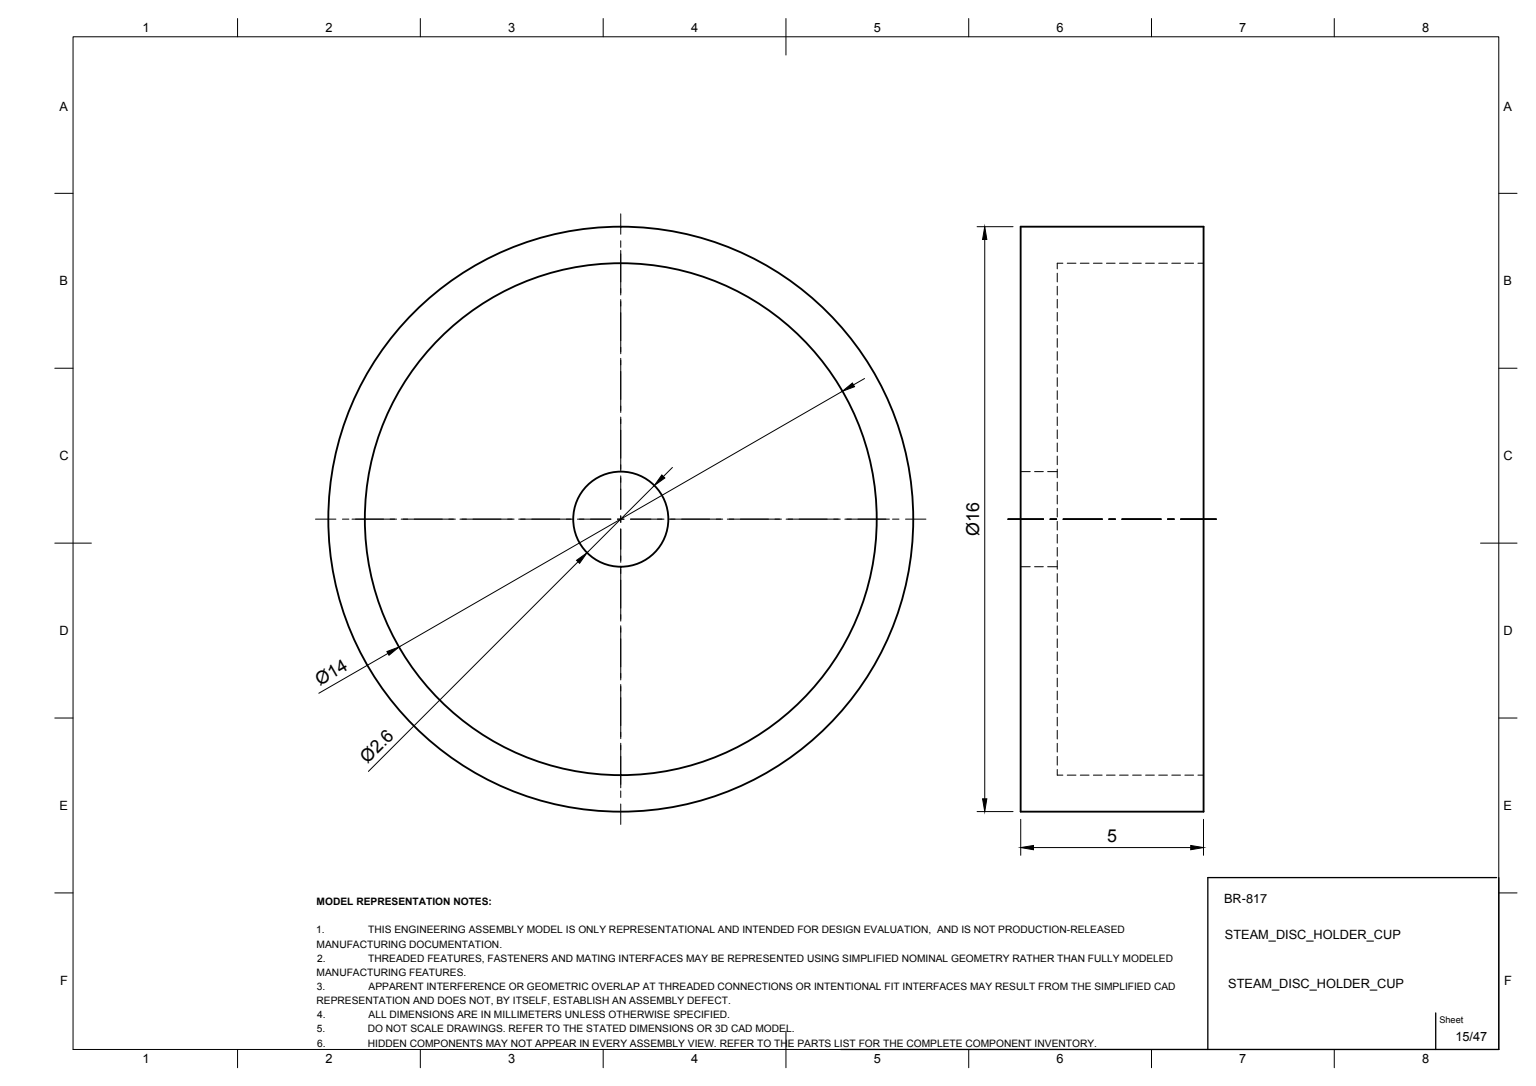
ISO-10303-21;
HEADER;
FILE_DESCRIPTION((''),'2;1');
FILE_NAME('STEAM_DISC_HOLDER_CUP.step','2026-10-01T22:07:29-07:00',(''),(''),'','','');
FILE_SCHEMA (('AUTOMOTIVE_DESIGN { 1 0 10303 214 3 1 1 }'));
ENDSEC;
DATA;
#10=MECHANICAL_DESIGN_GEOMETRIC_PRESENTATION_REPRESENTATION('',(#549),#15484);
#479=SHAPE_REPRESENTATION_RELATIONSHIP('SRR','None',#15628,#514) ;
#514=ADVANCED_BREP_SHAPE_REPRESENTATION('',(#591),#15452) ;
#549=STYLED_ITEM('',(#15834),#591) ;
#591=MANIFOLD_SOLID_BREP('STEAM_DISC_HOLDER_CUP',#8258) ;
#657=CYLINDRICAL_SURFACE('',#8871,0.13) ;
#658=CYLINDRICAL_SURFACE('',#8874,0.7) ;
#659=CYLINDRICAL_SURFACE('',#8879,0.8) ;
#849=FACE_BOUND('',#2016,.T.) ;
#850=FACE_BOUND('',#2019,.T.) ;
#851=FACE_BOUND('',#2021,.T.) ;
#948=CIRCLE('',#8872,0.13) ;
#949=CIRCLE('',#8873,0.13) ;
#950=CIRCLE('',#8875,0.7) ;
#951=CIRCLE('',#8876,0.7) ;
#952=CIRCLE('',#8878,0.8) ;
#953=CIRCLE('',#8880,0.8) ;
#1474=FACE_OUTER_BOUND('',#2013,.T.) ;
#1475=FACE_OUTER_BOUND('',#2014,.T.) ;
#1476=FACE_OUTER_BOUND('',#2015,.T.) ;
#1477=FACE_OUTER_BOUND('',#2017,.T.) ;
#1478=FACE_OUTER_BOUND('',#2018,.T.) ;
#1479=FACE_OUTER_BOUND('',#2020,.T.) ;
#2013=EDGE_LOOP('',(#5743,#5744,#5745,#5746)) ;
#2014=EDGE_LOOP('',(#5747,#5748,#5749,#5750)) ;
#2015=EDGE_LOOP('',(#5751)) ;
#2016=EDGE_LOOP('',(#5752)) ;
#2017=EDGE_LOOP('',(#5753,#5754,#5755,#5756)) ;
#2018=EDGE_LOOP('',(#5757)) ;
#2019=EDGE_LOOP('',(#5758)) ;
#2020=EDGE_LOOP('',(#5759)) ;
#2021=EDGE_LOOP('',(#5760)) ;
#2612=LINE('',#13407,#3086) ;
#2613=LINE('',#13413,#3087) ;
#2614=LINE('',#13420,#3088) ;
#3086=VECTOR('',#10479,0.13) ;
#3087=VECTOR('',#10486,0.7) ;
#3088=VECTOR('',#10495,0.8) ;
#3545=VERTEX_POINT('',#13404) ;
#3546=VERTEX_POINT('',#13406) ;
#3547=VERTEX_POINT('',#13410) ;
#3548=VERTEX_POINT('',#13412) ;
#3549=VERTEX_POINT('',#13416) ;
#3550=VERTEX_POINT('',#13419) ;
#4376=EDGE_CURVE('',#3545,#3545,#948,.T.) ;
#4377=EDGE_CURVE('',#3545,#3546,#2612,.T.) ;
#4378=EDGE_CURVE('',#3546,#3546,#949,.T.) ;
#4379=EDGE_CURVE('',#3547,#3547,#950,.T.) ;
#4380=EDGE_CURVE('',#3547,#3548,#2613,.T.) ;
#4381=EDGE_CURVE('',#3548,#3548,#951,.T.) ;
#4382=EDGE_CURVE('',#3549,#3549,#952,.T.) ;
#4383=EDGE_CURVE('',#3549,#3550,#2614,.T.) ;
#4384=EDGE_CURVE('',#3550,#3550,#953,.T.) ;
#5743=ORIENTED_EDGE('',*,*,#4376,.F.) ;
#5744=ORIENTED_EDGE('',*,*,#4377,.T.) ;
#5745=ORIENTED_EDGE('',*,*,#4378,.F.) ;
#5746=ORIENTED_EDGE('',*,*,#4377,.F.) ;
#5747=ORIENTED_EDGE('',*,*,#4379,.F.) ;
#5748=ORIENTED_EDGE('',*,*,#4380,.T.) ;
#5749=ORIENTED_EDGE('',*,*,#4381,.F.) ;
#5750=ORIENTED_EDGE('',*,*,#4380,.F.) ;
#5751=ORIENTED_EDGE('',*,*,#4382,.T.) ;
#5752=ORIENTED_EDGE('',*,*,#4381,.T.) ;
#5753=ORIENTED_EDGE('',*,*,#4382,.F.) ;
#5754=ORIENTED_EDGE('',*,*,#4383,.T.) ;
#5755=ORIENTED_EDGE('',*,*,#4384,.F.) ;
#5756=ORIENTED_EDGE('',*,*,#4383,.F.) ;
#5757=ORIENTED_EDGE('',*,*,#4384,.T.) ;
#5758=ORIENTED_EDGE('',*,*,#4376,.T.) ;
#5759=ORIENTED_EDGE('',*,*,#4379,.T.) ;
#5760=ORIENTED_EDGE('',*,*,#4378,.T.) ;
#7614=PLANE('',#8877) ;
#7615=PLANE('',#8881) ;
#7616=PLANE('',#8882) ;
#7861=ADVANCED_FACE('',(#1474),#657,.F.) ;
#7862=ADVANCED_FACE('',(#1475),#658,.F.) ;
#7863=ADVANCED_FACE('',(#1476,#849),#7614,.T.) ;
#7864=ADVANCED_FACE('',(#1477),#659,.T.) ;
#7865=ADVANCED_FACE('',(#1478,#850),#7615,.T.) ;
#7866=ADVANCED_FACE('',(#1479,#851),#7616,.T.) ;
#8258=CLOSED_SHELL('',(#7861,#7862,#7863,#7864,#7865,#7866)) ;
#8870=AXIS2_PLACEMENT_3D('',#13402,#10473,#10474) ;
#8871=AXIS2_PLACEMENT_3D('',#13403,#10475,#10476) ;
#8872=AXIS2_PLACEMENT_3D('',#13405,#10477,#10478) ;
#8873=AXIS2_PLACEMENT_3D('',#13408,#10480,#10481) ;
#8874=AXIS2_PLACEMENT_3D('',#13409,#10482,#10483) ;
#8875=AXIS2_PLACEMENT_3D('',#13411,#10484,#10485) ;
#8876=AXIS2_PLACEMENT_3D('',#13414,#10487,#10488) ;
#8877=AXIS2_PLACEMENT_3D('',#13415,#10489,#10490) ;
#8878=AXIS2_PLACEMENT_3D('',#13417,#10491,#10492) ;
#8879=AXIS2_PLACEMENT_3D('',#13418,#10493,#10494) ;
#8880=AXIS2_PLACEMENT_3D('',#13421,#10496,#10497) ;
#8881=AXIS2_PLACEMENT_3D('',#13422,#10498,#10499) ;
#8882=AXIS2_PLACEMENT_3D('',#13423,#10500,#10501) ;
#10473=DIRECTION('axis',(0.,0.,1.)) ;
#10474=DIRECTION('refdir',(1.,0.,0.)) ;
#10475=DIRECTION('center_axis',(0.,0.,1.)) ;
#10476=DIRECTION('ref_axis',(1.,0.,0.)) ;
#10477=DIRECTION('center_axis',(0.,0.,1.)) ;
#10478=DIRECTION('ref_axis',(1.,0.,0.)) ;
#10479=DIRECTION('',(0.,0.,1.)) ;
#10480=DIRECTION('center_axis',(0.,0.,-1.)) ;
#10481=DIRECTION('ref_axis',(1.,0.,0.)) ;
#10482=DIRECTION('center_axis',(0.,0.,1.)) ;
#10483=DIRECTION('ref_axis',(1.,0.,0.)) ;
#10484=DIRECTION('center_axis',(0.,0.,1.)) ;
#10485=DIRECTION('ref_axis',(1.,0.,0.)) ;
#10486=DIRECTION('',(0.,0.,1.)) ;
#10487=DIRECTION('center_axis',(0.,0.,-1.)) ;
#10488=DIRECTION('ref_axis',(1.,0.,0.)) ;
#10489=DIRECTION('center_axis',(0.,0.,1.)) ;
#10490=DIRECTION('ref_axis',(1.,0.,0.)) ;
#10491=DIRECTION('center_axis',(0.,0.,1.)) ;
#10492=DIRECTION('ref_axis',(1.,0.,0.)) ;
#10493=DIRECTION('center_axis',(0.,0.,1.)) ;
#10494=DIRECTION('ref_axis',(1.,0.,0.)) ;
#10495=DIRECTION('',(0.,0.,-1.)) ;
#10496=DIRECTION('center_axis',(0.,0.,-1.)) ;
#10497=DIRECTION('ref_axis',(1.,0.,0.)) ;
#10498=DIRECTION('center_axis',(0.,0.,-1.)) ;
#10499=DIRECTION('ref_axis',(-1.,0.,0.)) ;
#10500=DIRECTION('center_axis',(0.,0.,1.)) ;
#10501=DIRECTION('ref_axis',(1.,0.,0.)) ;
#13402=CARTESIAN_POINT('',(0.,0.,0.)) ;
#13403=CARTESIAN_POINT('Origin',(2.,0.8,0.75)) ;
#13404=CARTESIAN_POINT('',(1.87,0.8,0.7)) ;
#13405=CARTESIAN_POINT('Origin',(2.,0.8,0.7)) ;
#13406=CARTESIAN_POINT('',(1.87,0.8,0.8)) ;
#13407=CARTESIAN_POINT('',(1.87,0.8,0.75)) ;
#13408=CARTESIAN_POINT('Origin',(2.,0.8,0.8)) ;
#13409=CARTESIAN_POINT('Origin',(2.,0.8,1.)) ;
#13410=CARTESIAN_POINT('',(1.3,0.8,0.8)) ;
#13411=CARTESIAN_POINT('Origin',(2.,0.8,0.8)) ;
#13412=CARTESIAN_POINT('',(1.3,0.8,1.2)) ;
#13413=CARTESIAN_POINT('',(1.3,0.8,1.)) ;
#13414=CARTESIAN_POINT('Origin',(2.,0.8,1.2)) ;
#13415=CARTESIAN_POINT('Origin',(2.,0.8,1.2)) ;
#13416=CARTESIAN_POINT('',(1.2,0.8,1.2)) ;
#13417=CARTESIAN_POINT('Origin',(2.,0.8,1.2)) ;
#13418=CARTESIAN_POINT('Origin',(2.,0.8,0.75)) ;
#13419=CARTESIAN_POINT('',(1.2,0.8,0.7)) ;
#13420=CARTESIAN_POINT('',(1.2,0.8,0.75)) ;
#13421=CARTESIAN_POINT('Origin',(2.,0.8,0.7)) ;
#13422=CARTESIAN_POINT('Origin',(2.,0.8,0.7)) ;
#13423=CARTESIAN_POINT('Origin',(2.,0.8,0.8)) ;
#15409=UNCERTAINTY_MEASURE_WITH_UNIT(LENGTH_MEASURE(0.001),#15485,
'DISTANCE_ACCURACY_VALUE',
'Maximum model space distance between geometric entities at asserted c
onnectivities') ;
#15441=UNCERTAINTY_MEASURE_WITH_UNIT(LENGTH_MEASURE(0.001),#15485,
'DISTANCE_ACCURACY_VALUE',
'Maximum model space distance between geometric entities at asserted c
onnectivities') ;
#15452=(
GEOMETRIC_REPRESENTATION_CONTEXT(3)
GLOBAL_UNCERTAINTY_ASSIGNED_CONTEXT((#15409))
GLOBAL_UNIT_ASSIGNED_CONTEXT((#15485,#15487,#15488))
REPRESENTATION_CONTEXT('','3D')
) ;
#15484=(
GEOMETRIC_REPRESENTATION_CONTEXT(3)
GLOBAL_UNCERTAINTY_ASSIGNED_CONTEXT((#15441))
GLOBAL_UNIT_ASSIGNED_CONTEXT((#15485,#15487,#15488))
REPRESENTATION_CONTEXT('','3D')
) ;
#15485=(
LENGTH_UNIT()
NAMED_UNIT(*)
SI_UNIT(.CENTI.,.METRE.)
) ;
#15487=(
NAMED_UNIT(*)
PLANE_ANGLE_UNIT()
SI_UNIT($,.RADIAN.)
) ;
#15488=(
NAMED_UNIT(*)
SI_UNIT($,.STERADIAN.)
SOLID_ANGLE_UNIT()
) ;
#15499=SHAPE_DEFINITION_REPRESENTATION(#15547,#15628) ;
#15547=PRODUCT_DEFINITION_SHAPE('',$,#15671) ;
#15628=SHAPE_REPRESENTATION('',(#8870),#15452) ;
#15660=PRODUCT_DEFINITION_CONTEXT('part definition',#15788,'design') ;
#15671=PRODUCT_DEFINITION('STEAM_DISC_HOLDER_CUP',
'STEAM_DISC_HOLDER_CUP',#15713,#15660) ;
#15713=PRODUCT_DEFINITION_FORMATION('',$,#15800) ;
#15788=APPLICATION_CONTEXT(
'Core Data for Automotive Mechanical Design Process') ;
#15789=PRODUCT_CONTEXT('part definition',#15788,'mechanical') ;
#15800=PRODUCT('STEAM_DISC_HOLDER_CUP','STEAM_DISC_HOLDER_CUP',$,(#15789)) ;
#15834=PRESENTATION_STYLE_ASSIGNMENT((#15846)) ;
#15846=SURFACE_STYLE_USAGE(.BOTH.,#15858) ;
#15858=SURFACE_SIDE_STYLE('',(#15870)) ;
#15870=SURFACE_STYLE_FILL_AREA(#15882) ;
#15882=FILL_AREA_STYLE('Brass - Polished',(#15894)) ;
#15894=FILL_AREA_STYLE_COLOUR('Brass - Polished',#15906) ;
#15906=COLOUR_RGB('Brass - Polished', 0.08235294, 0.09019608, 0.10196078) ;
ENDSEC;
END-ISO-10303-21;
